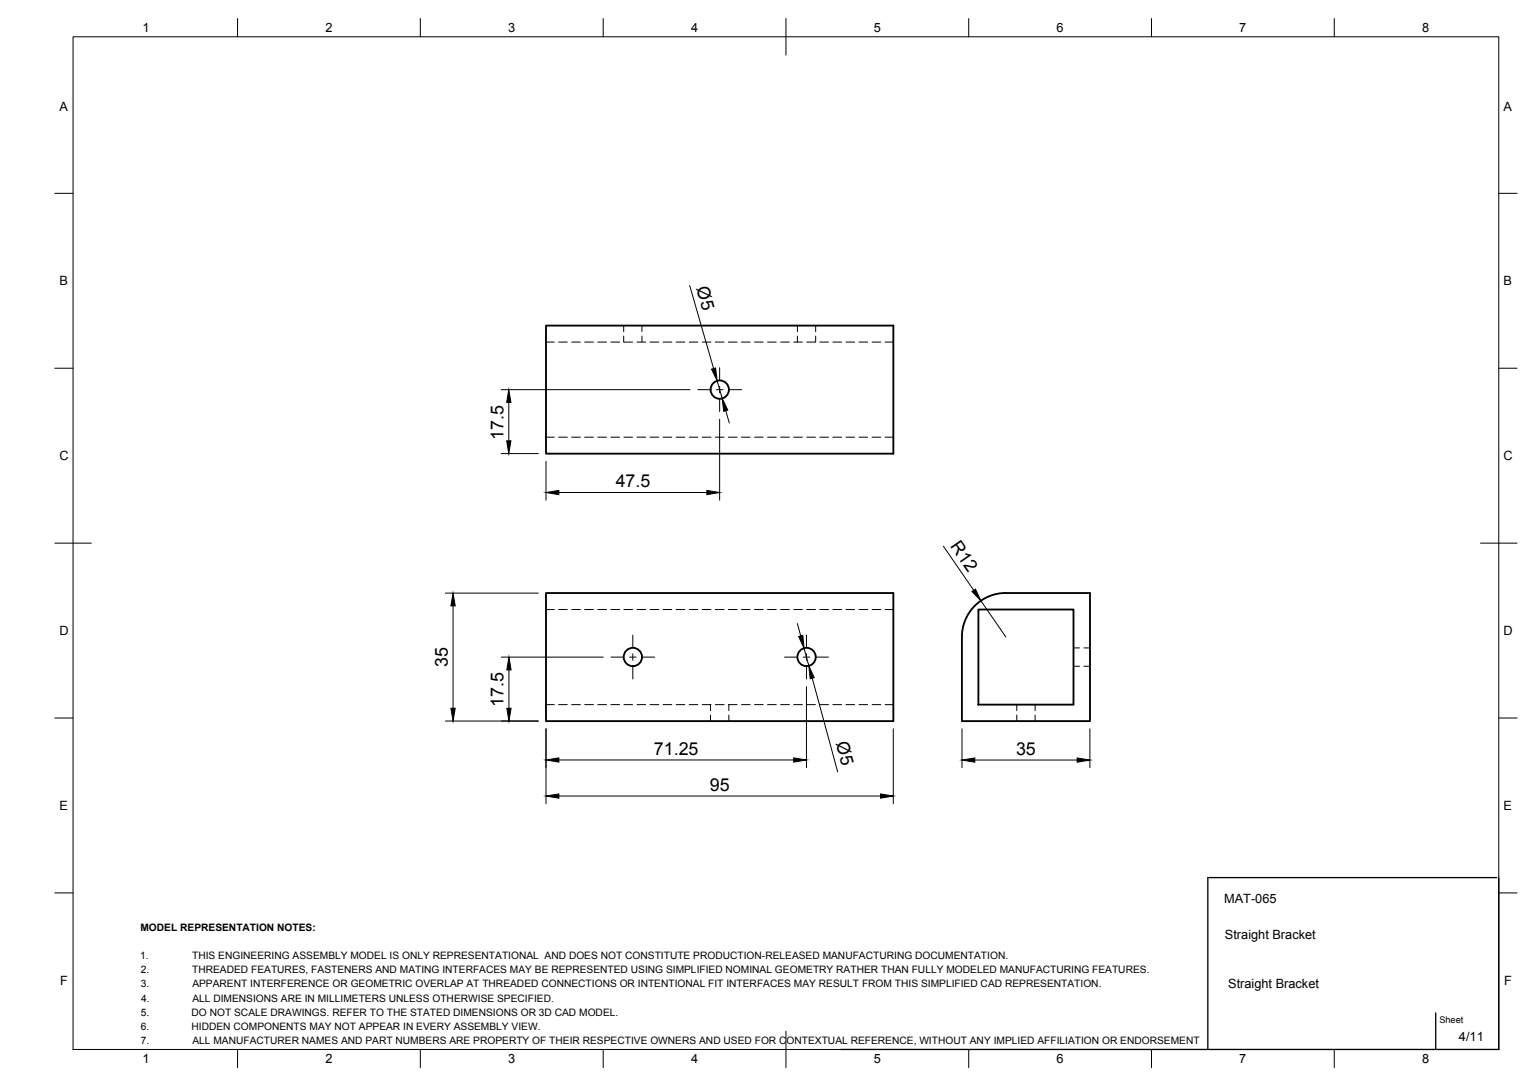
ISO-10303-21;
HEADER;
/* Generated by software containing ST-Developer
 * from STEP Tools, Inc. (www.steptools.com) 
 */

FILE_DESCRIPTION(
/* description */ (
'CAx-IF Rec.Pracs.---Representation and Presentation of Product Manufa
cturing Information (PMI)---4.0---2014-10-13'),
/* implementation_level */ '2;1');

FILE_NAME(
/* name */ 'Straight Bracket.step',
/* time_stamp */ '2026-11-15T23:28:27-08:00',
/* author */ (''),
/* organization */ (''),
/* preprocessor_version */ 'ST-DEVELOPER v20.2',
/* originating_system */ 'Autodesk Translation Framework v15.17.0.0',
/* authorisation */ '');

FILE_SCHEMA (('AUTOMOTIVE_DESIGN { 1 0 10303 214 3 1 1 }'));
ENDSEC;

DATA;
#10=MECHANICAL_DESIGN_GEOMETRIC_PRESENTATION_REPRESENTATION('',(#192),#7756);
#174=SHAPE_REPRESENTATION_RELATIONSHIP('SRR','None',#7822,#183);
#183=ADVANCED_BREP_SHAPE_REPRESENTATION('',(#201),#7750);
#192=STYLED_ITEM('',(#7876),#201);
#201=MANIFOLD_SOLID_BREP('Body1',#4629);
#216=CYLINDRICAL_SURFACE('',#4809,0.012);
#217=CYLINDRICAL_SURFACE('',#4817,0.0025);
#218=CYLINDRICAL_SURFACE('',#4818,0.0025);
#219=CYLINDRICAL_SURFACE('',#4819,0.0025);
#282=CIRCLE('',#4799,0.012);
#283=CIRCLE('',#4801,0.012);
#284=CIRCLE('',#4803,0.0025);
#285=CIRCLE('',#4806,0.0025);
#286=CIRCLE('',#4807,0.0025);
#287=CIRCLE('',#4811,0.0025);
#288=CIRCLE('',#4812,0.0025);
#289=CIRCLE('',#4814,0.0025);
#397=FACE_BOUND('',#745,.T.);
#398=FACE_BOUND('',#747,.T.);
#399=FACE_BOUND('',#749,.T.);
#400=FACE_BOUND('',#752,.T.);
#401=FACE_BOUND('',#753,.T.);
#402=FACE_BOUND('',#757,.T.);
#403=FACE_BOUND('',#758,.T.);
#404=FACE_BOUND('',#760,.T.);
#492=FACE_OUTER_BOUND('',#744,.T.);
#493=FACE_OUTER_BOUND('',#746,.T.);
#494=FACE_OUTER_BOUND('',#748,.T.);
#495=FACE_OUTER_BOUND('',#750,.T.);
#496=FACE_OUTER_BOUND('',#751,.T.);
#497=FACE_OUTER_BOUND('',#754,.T.);
#498=FACE_OUTER_BOUND('',#755,.T.);
#499=FACE_OUTER_BOUND('',#756,.T.);
#500=FACE_OUTER_BOUND('',#759,.T.);
#501=FACE_OUTER_BOUND('',#761,.T.);
#502=FACE_OUTER_BOUND('',#762,.T.);
#503=FACE_OUTER_BOUND('',#763,.T.);
#504=FACE_OUTER_BOUND('',#764,.T.);
#505=FACE_OUTER_BOUND('',#765,.T.);
#744=EDGE_LOOP('',(#3191,#3192,#3193,#3194,#3195));
#745=EDGE_LOOP('',(#3196,#3197,#3198,#3199));
#746=EDGE_LOOP('',(#3200,#3201,#3202,#3203,#3204));
#747=EDGE_LOOP('',(#3205,#3206,#3207,#3208));
#748=EDGE_LOOP('',(#3209,#3210,#3211,#3212));
#749=EDGE_LOOP('',(#3213));
#750=EDGE_LOOP('',(#3214,#3215,#3216,#3217));
#751=EDGE_LOOP('',(#3218,#3219,#3220,#3221));
#752=EDGE_LOOP('',(#3222));
#753=EDGE_LOOP('',(#3223));
#754=EDGE_LOOP('',(#3224,#3225,#3226,#3227));
#755=EDGE_LOOP('',(#3228,#3229,#3230,#3231));
#756=EDGE_LOOP('',(#3232,#3233,#3234,#3235));
#757=EDGE_LOOP('',(#3236));
#758=EDGE_LOOP('',(#3237));
#759=EDGE_LOOP('',(#3238,#3239,#3240,#3241));
#760=EDGE_LOOP('',(#3242));
#761=EDGE_LOOP('',(#3243,#3244,#3245,#3246));
#762=EDGE_LOOP('',(#3247,#3248,#3249,#3250));
#763=EDGE_LOOP('',(#3251,#3252,#3253,#3254));
#764=EDGE_LOOP('',(#3255,#3256,#3257,#3258));
#765=EDGE_LOOP('',(#3259,#3260,#3261,#3262));
#1073=LINE('',#6632,#1566);
#1074=LINE('',#6636,#1567);
#1075=LINE('',#6638,#1568);
#1076=LINE('',#6639,#1569);
#1077=LINE('',#6642,#1570);
#1078=LINE('',#6644,#1571);
#1079=LINE('',#6646,#1572);
#1080=LINE('',#6647,#1573);
#1081=LINE('',#6651,#1574);
#1082=LINE('',#6655,#1575);
#1083=LINE('',#6657,#1576);
#1084=LINE('',#6658,#1577);
#1085=LINE('',#6661,#1578);
#1086=LINE('',#6663,#1579);
#1087=LINE('',#6665,#1580);
#1088=LINE('',#6666,#1581);
#1089=LINE('',#6668,#1582);
#1090=LINE('',#6669,#1583);
#1091=LINE('',#6673,#1584);
#1092=LINE('',#6674,#1585);
#1093=LINE('',#6681,#1586);
#1094=LINE('',#6684,#1587);
#1095=LINE('',#6685,#1588);
#1096=LINE('',#6691,#1589);
#1097=LINE('',#6695,#1590);
#1098=LINE('',#6698,#1591);
#1099=LINE('',#6700,#1592);
#1100=LINE('',#6702,#1593);
#1566=VECTOR('',#5341,1.);
#1567=VECTOR('',#5344,1.);
#1568=VECTOR('',#5345,1.);
#1569=VECTOR('',#5346,1.);
#1570=VECTOR('',#5347,1.);
#1571=VECTOR('',#5348,1.);
#1572=VECTOR('',#5349,1.);
#1573=VECTOR('',#5350,1.);
#1574=VECTOR('',#5353,1.);
#1575=VECTOR('',#5356,1.);
#1576=VECTOR('',#5357,1.);
#1577=VECTOR('',#5358,1.);
#1578=VECTOR('',#5359,1.);
#1579=VECTOR('',#5360,1.);
#1580=VECTOR('',#5361,1.);
#1581=VECTOR('',#5362,1.);
#1582=VECTOR('',#5365,1.);
#1583=VECTOR('',#5366,1.);
#1584=VECTOR('',#5371,1.);
#1585=VECTOR('',#5372,1.);
#1586=VECTOR('',#5381,1.);
#1587=VECTOR('',#5386,1.);
#1588=VECTOR('',#5387,1.);
#1589=VECTOR('',#5394,1.);
#1590=VECTOR('',#5399,1.);
#1591=VECTOR('',#5404,0.0025);
#1592=VECTOR('',#5407,0.0025);
#1593=VECTOR('',#5410,0.0025);
#2044=VERTEX_POINT('',#6630);
#2045=VERTEX_POINT('',#6631);
#2046=VERTEX_POINT('',#6633);
#2047=VERTEX_POINT('',#6635);
#2048=VERTEX_POINT('',#6637);
#2049=VERTEX_POINT('',#6640);
#2050=VERTEX_POINT('',#6641);
#2051=VERTEX_POINT('',#6643);
#2052=VERTEX_POINT('',#6645);
#2053=VERTEX_POINT('',#6649);
#2054=VERTEX_POINT('',#6650);
#2055=VERTEX_POINT('',#6652);
#2056=VERTEX_POINT('',#6654);
#2057=VERTEX_POINT('',#6656);
#2058=VERTEX_POINT('',#6659);
#2059=VERTEX_POINT('',#6660);
#2060=VERTEX_POINT('',#6662);
#2061=VERTEX_POINT('',#6664);
#2062=VERTEX_POINT('',#6670);
#2063=VERTEX_POINT('',#6676);
#2064=VERTEX_POINT('',#6678);
#2065=VERTEX_POINT('',#6686);
#2066=VERTEX_POINT('',#6688);
#2067=VERTEX_POINT('',#6692);
#2479=EDGE_CURVE('',#2044,#2045,#1073,.T.);
#2480=EDGE_CURVE('',#2045,#2046,#282,.F.);
#2481=EDGE_CURVE('',#2047,#2046,#1074,.T.);
#2482=EDGE_CURVE('',#2048,#2047,#1075,.T.);
#2483=EDGE_CURVE('',#2048,#2044,#1076,.T.);
#2484=EDGE_CURVE('',#2049,#2050,#1077,.T.);
#2485=EDGE_CURVE('',#2050,#2051,#1078,.T.);
#2486=EDGE_CURVE('',#2052,#2051,#1079,.T.);
#2487=EDGE_CURVE('',#2049,#2052,#1080,.T.);
#2488=EDGE_CURVE('',#2053,#2054,#1081,.T.);
#2489=EDGE_CURVE('',#2054,#2055,#283,.T.);
#2490=EDGE_CURVE('',#2056,#2055,#1082,.T.);
#2491=EDGE_CURVE('',#2057,#2056,#1083,.T.);
#2492=EDGE_CURVE('',#2057,#2053,#1084,.T.);
#2493=EDGE_CURVE('',#2058,#2059,#1085,.T.);
#2494=EDGE_CURVE('',#2059,#2060,#1086,.T.);
#2495=EDGE_CURVE('',#2061,#2060,#1087,.T.);
#2496=EDGE_CURVE('',#2058,#2061,#1088,.T.);
#2497=EDGE_CURVE('',#2044,#2056,#1089,.T.);
#2498=EDGE_CURVE('',#2048,#2057,#1090,.T.);
#2499=EDGE_CURVE('',#2062,#2062,#284,.T.);
#2500=EDGE_CURVE('',#2046,#2054,#1091,.T.);
#2501=EDGE_CURVE('',#2047,#2053,#1092,.T.);
#2502=EDGE_CURVE('',#2063,#2063,#285,.T.);
#2503=EDGE_CURVE('',#2064,#2064,#286,.T.);
#2504=EDGE_CURVE('',#2055,#2045,#1093,.F.);
#2505=EDGE_CURVE('',#2059,#2050,#1094,.T.);
#2506=EDGE_CURVE('',#2060,#2049,#1095,.T.);
#2507=EDGE_CURVE('',#2065,#2065,#287,.T.);
#2508=EDGE_CURVE('',#2066,#2066,#288,.T.);
#2509=EDGE_CURVE('',#2061,#2052,#1096,.T.);
#2510=EDGE_CURVE('',#2067,#2067,#289,.T.);
#2511=EDGE_CURVE('',#2058,#2051,#1097,.T.);
#2512=EDGE_CURVE('',#2067,#2062,#1098,.T.);
#2513=EDGE_CURVE('',#2066,#2064,#1099,.T.);
#2514=EDGE_CURVE('',#2065,#2063,#1100,.T.);
#3191=ORIENTED_EDGE('',*,*,#2479,.T.);
#3192=ORIENTED_EDGE('',*,*,#2480,.T.);
#3193=ORIENTED_EDGE('',*,*,#2481,.F.);
#3194=ORIENTED_EDGE('',*,*,#2482,.F.);
#3195=ORIENTED_EDGE('',*,*,#2483,.T.);
#3196=ORIENTED_EDGE('',*,*,#2484,.T.);
#3197=ORIENTED_EDGE('',*,*,#2485,.T.);
#3198=ORIENTED_EDGE('',*,*,#2486,.F.);
#3199=ORIENTED_EDGE('',*,*,#2487,.F.);
#3200=ORIENTED_EDGE('',*,*,#2488,.T.);
#3201=ORIENTED_EDGE('',*,*,#2489,.T.);
#3202=ORIENTED_EDGE('',*,*,#2490,.F.);
#3203=ORIENTED_EDGE('',*,*,#2491,.F.);
#3204=ORIENTED_EDGE('',*,*,#2492,.T.);
#3205=ORIENTED_EDGE('',*,*,#2493,.T.);
#3206=ORIENTED_EDGE('',*,*,#2494,.T.);
#3207=ORIENTED_EDGE('',*,*,#2495,.F.);
#3208=ORIENTED_EDGE('',*,*,#2496,.F.);
#3209=ORIENTED_EDGE('',*,*,#2497,.F.);
#3210=ORIENTED_EDGE('',*,*,#2483,.F.);
#3211=ORIENTED_EDGE('',*,*,#2498,.T.);
#3212=ORIENTED_EDGE('',*,*,#2491,.T.);
#3213=ORIENTED_EDGE('',*,*,#2499,.F.);
#3214=ORIENTED_EDGE('',*,*,#2481,.T.);
#3215=ORIENTED_EDGE('',*,*,#2500,.T.);
#3216=ORIENTED_EDGE('',*,*,#2488,.F.);
#3217=ORIENTED_EDGE('',*,*,#2501,.F.);
#3218=ORIENTED_EDGE('',*,*,#2498,.F.);
#3219=ORIENTED_EDGE('',*,*,#2482,.T.);
#3220=ORIENTED_EDGE('',*,*,#2501,.T.);
#3221=ORIENTED_EDGE('',*,*,#2492,.F.);
#3222=ORIENTED_EDGE('',*,*,#2502,.F.);
#3223=ORIENTED_EDGE('',*,*,#2503,.F.);
#3224=ORIENTED_EDGE('',*,*,#2490,.T.);
#3225=ORIENTED_EDGE('',*,*,#2504,.T.);
#3226=ORIENTED_EDGE('',*,*,#2479,.F.);
#3227=ORIENTED_EDGE('',*,*,#2497,.T.);
#3228=ORIENTED_EDGE('',*,*,#2480,.F.);
#3229=ORIENTED_EDGE('',*,*,#2504,.F.);
#3230=ORIENTED_EDGE('',*,*,#2489,.F.);
#3231=ORIENTED_EDGE('',*,*,#2500,.F.);
#3232=ORIENTED_EDGE('',*,*,#2505,.T.);
#3233=ORIENTED_EDGE('',*,*,#2484,.F.);
#3234=ORIENTED_EDGE('',*,*,#2506,.F.);
#3235=ORIENTED_EDGE('',*,*,#2494,.F.);
#3236=ORIENTED_EDGE('',*,*,#2507,.F.);
#3237=ORIENTED_EDGE('',*,*,#2508,.F.);
#3238=ORIENTED_EDGE('',*,*,#2495,.T.);
#3239=ORIENTED_EDGE('',*,*,#2506,.T.);
#3240=ORIENTED_EDGE('',*,*,#2487,.T.);
#3241=ORIENTED_EDGE('',*,*,#2509,.F.);
#3242=ORIENTED_EDGE('',*,*,#2510,.T.);
#3243=ORIENTED_EDGE('',*,*,#2496,.T.);
#3244=ORIENTED_EDGE('',*,*,#2509,.T.);
#3245=ORIENTED_EDGE('',*,*,#2486,.T.);
#3246=ORIENTED_EDGE('',*,*,#2511,.F.);
#3247=ORIENTED_EDGE('',*,*,#2511,.T.);
#3248=ORIENTED_EDGE('',*,*,#2485,.F.);
#3249=ORIENTED_EDGE('',*,*,#2505,.F.);
#3250=ORIENTED_EDGE('',*,*,#2493,.F.);
#3251=ORIENTED_EDGE('',*,*,#2510,.F.);
#3252=ORIENTED_EDGE('',*,*,#2512,.T.);
#3253=ORIENTED_EDGE('',*,*,#2499,.T.);
#3254=ORIENTED_EDGE('',*,*,#2512,.F.);
#3255=ORIENTED_EDGE('',*,*,#2508,.T.);
#3256=ORIENTED_EDGE('',*,*,#2513,.T.);
#3257=ORIENTED_EDGE('',*,*,#2503,.T.);
#3258=ORIENTED_EDGE('',*,*,#2513,.F.);
#3259=ORIENTED_EDGE('',*,*,#2507,.T.);
#3260=ORIENTED_EDGE('',*,*,#2514,.T.);
#3261=ORIENTED_EDGE('',*,*,#2502,.T.);
#3262=ORIENTED_EDGE('',*,*,#2514,.F.);
#4250=PLANE('',#4798);
#4251=PLANE('',#4800);
#4252=PLANE('',#4802);
#4253=PLANE('',#4804);
#4254=PLANE('',#4805);
#4255=PLANE('',#4808);
#4256=PLANE('',#4810);
#4257=PLANE('',#4813);
#4258=PLANE('',#4815);
#4259=PLANE('',#4816);
#4433=ADVANCED_FACE('',(#492,#397),#4250,.F.);
#4434=ADVANCED_FACE('',(#493,#398),#4251,.T.);
#4435=ADVANCED_FACE('',(#494,#399),#4252,.T.);
#4436=ADVANCED_FACE('',(#495),#4253,.F.);
#4437=ADVANCED_FACE('',(#496,#400,#401),#4254,.T.);
#4438=ADVANCED_FACE('',(#497),#4255,.F.);
#4439=ADVANCED_FACE('',(#498),#216,.T.);
#4440=ADVANCED_FACE('',(#499,#402,#403),#4256,.T.);
#4441=ADVANCED_FACE('',(#500,#404),#4257,.F.);
#4442=ADVANCED_FACE('',(#501),#4258,.F.);
#4443=ADVANCED_FACE('',(#502),#4259,.T.);
#4444=ADVANCED_FACE('',(#503),#217,.F.);
#4445=ADVANCED_FACE('',(#504),#218,.F.);
#4446=ADVANCED_FACE('',(#505),#219,.F.);
#4629=CLOSED_SHELL('',(#4433,#4434,#4435,#4436,#4437,#4438,#4439,#4440,
#4441,#4442,#4443,#4444,#4445,#4446));
#4797=AXIS2_PLACEMENT_3D('',#6628,#5337,#5338);
#4798=AXIS2_PLACEMENT_3D('',#6629,#5339,#5340);
#4799=AXIS2_PLACEMENT_3D('',#6634,#5342,#5343);
#4800=AXIS2_PLACEMENT_3D('',#6648,#5351,#5352);
#4801=AXIS2_PLACEMENT_3D('',#6653,#5354,#5355);
#4802=AXIS2_PLACEMENT_3D('',#6667,#5363,#5364);
#4803=AXIS2_PLACEMENT_3D('',#6671,#5367,#5368);
#4804=AXIS2_PLACEMENT_3D('',#6672,#5369,#5370);
#4805=AXIS2_PLACEMENT_3D('',#6675,#5373,#5374);
#4806=AXIS2_PLACEMENT_3D('',#6677,#5375,#5376);
#4807=AXIS2_PLACEMENT_3D('',#6679,#5377,#5378);
#4808=AXIS2_PLACEMENT_3D('',#6680,#5379,#5380);
#4809=AXIS2_PLACEMENT_3D('',#6682,#5382,#5383);
#4810=AXIS2_PLACEMENT_3D('',#6683,#5384,#5385);
#4811=AXIS2_PLACEMENT_3D('',#6687,#5388,#5389);
#4812=AXIS2_PLACEMENT_3D('',#6689,#5390,#5391);
#4813=AXIS2_PLACEMENT_3D('',#6690,#5392,#5393);
#4814=AXIS2_PLACEMENT_3D('',#6693,#5395,#5396);
#4815=AXIS2_PLACEMENT_3D('',#6694,#5397,#5398);
#4816=AXIS2_PLACEMENT_3D('',#6696,#5400,#5401);
#4817=AXIS2_PLACEMENT_3D('',#6697,#5402,#5403);
#4818=AXIS2_PLACEMENT_3D('',#6699,#5405,#5406);
#4819=AXIS2_PLACEMENT_3D('',#6701,#5408,#5409);
#5337=DIRECTION('axis',(0.,0.,1.));
#5338=DIRECTION('refdir',(1.,0.,0.));
#5339=DIRECTION('center_axis',(1.,0.,0.));
#5340=DIRECTION('ref_axis',(0.,0.,-1.));
#5341=DIRECTION('',(0.,-1.,0.));
#5342=DIRECTION('center_axis',(1.,0.,0.));
#5343=DIRECTION('ref_axis',(0.,0.,-1.));
#5344=DIRECTION('',(0.,0.,-1.));
#5345=DIRECTION('',(0.,-1.,0.));
#5346=DIRECTION('',(0.,0.,-1.));
#5347=DIRECTION('',(0.,-1.,0.));
#5348=DIRECTION('',(0.,0.,-1.));
#5349=DIRECTION('',(0.,-1.,0.));
#5350=DIRECTION('',(0.,-6.67201336914157E-17,-1.));
#5351=DIRECTION('center_axis',(1.,0.,0.));
#5352=DIRECTION('ref_axis',(0.,0.,-1.));
#5353=DIRECTION('',(0.,0.,-1.));
#5354=DIRECTION('center_axis',(1.,0.,0.));
#5355=DIRECTION('ref_axis',(0.,0.,-1.));
#5356=DIRECTION('',(0.,-1.,0.));
#5357=DIRECTION('',(0.,0.,-1.));
#5358=DIRECTION('',(0.,-1.,0.));
#5359=DIRECTION('',(0.,0.,1.));
#5360=DIRECTION('',(0.,1.,0.));
#5361=DIRECTION('',(0.,6.67201336914157E-17,1.));
#5362=DIRECTION('',(0.,1.,0.));
#5363=DIRECTION('center_axis',(-1.82602471155453E-16,1.,0.));
#5364=DIRECTION('ref_axis',(-1.,-1.82602471155453E-16,0.));
#5365=DIRECTION('',(1.,1.82602471155453E-16,0.));
#5366=DIRECTION('',(1.,1.82602471155453E-16,0.));
#5367=DIRECTION('center_axis',(-1.82602471155453E-16,1.,0.));
#5368=DIRECTION('ref_axis',(-1.,-1.82602471155453E-16,0.));
#5369=DIRECTION('center_axis',(-2.19122965386544E-16,1.,0.));
#5370=DIRECTION('ref_axis',(-1.,-2.19122965386544E-16,0.));
#5371=DIRECTION('',(1.,2.19122965386544E-16,0.));
#5372=DIRECTION('',(1.,2.19122965386544E-16,0.));
#5373=DIRECTION('center_axis',(0.,0.,1.));
#5374=DIRECTION('ref_axis',(1.,0.,0.));
#5375=DIRECTION('center_axis',(0.,0.,1.));
#5376=DIRECTION('ref_axis',(1.,0.,0.));
#5377=DIRECTION('center_axis',(0.,0.,1.));
#5378=DIRECTION('ref_axis',(1.,0.,0.));
#5379=DIRECTION('center_axis',(0.,0.,1.));
#5380=DIRECTION('ref_axis',(1.,0.,0.));
#5381=DIRECTION('',(1.,2.19122965386544E-16,0.));
#5382=DIRECTION('center_axis',(1.,2.19122965386544E-16,0.));
#5383=DIRECTION('ref_axis',(-2.19122965386544E-16,1.,0.));
#5384=DIRECTION('center_axis',(0.,0.,-1.));
#5385=DIRECTION('ref_axis',(-1.,0.,0.));
#5386=DIRECTION('',(-1.,0.,0.));
#5387=DIRECTION('',(-1.,0.,0.));
#5388=DIRECTION('center_axis',(0.,0.,-1.));
#5389=DIRECTION('ref_axis',(-1.,0.,0.));
#5390=DIRECTION('center_axis',(0.,0.,-1.));
#5391=DIRECTION('ref_axis',(-1.,0.,0.));
#5392=DIRECTION('center_axis',(0.,1.,-6.67201336914157E-17));
#5393=DIRECTION('ref_axis',(0.,6.67201336914157E-17,1.));
#5394=DIRECTION('',(-1.,0.,0.));
#5395=DIRECTION('center_axis',(0.,1.,-6.67201336914157E-17));
#5396=DIRECTION('ref_axis',(0.,6.67201336914157E-17,1.));
#5397=DIRECTION('center_axis',(0.,0.,-1.));
#5398=DIRECTION('ref_axis',(-1.,0.,0.));
#5399=DIRECTION('',(-1.,0.,0.));
#5400=DIRECTION('center_axis',(0.,1.,0.));
#5401=DIRECTION('ref_axis',(0.,0.,1.));
#5402=DIRECTION('center_axis',(-1.82602471155453E-16,1.,0.));
#5403=DIRECTION('ref_axis',(-1.,-1.82602471155453E-16,0.));
#5404=DIRECTION('',(-1.82602471155453E-16,1.,0.));
#5405=DIRECTION('center_axis',(0.,0.,1.));
#5406=DIRECTION('ref_axis',(1.,0.,0.));
#5407=DIRECTION('',(0.,0.,1.));
#5408=DIRECTION('center_axis',(0.,0.,1.));
#5409=DIRECTION('ref_axis',(1.,0.,0.));
#5410=DIRECTION('',(0.,0.,1.));
#6628=CARTESIAN_POINT('',(0.,0.,0.));
#6629=CARTESIAN_POINT('Origin',(-0.0475,-1.04083408558608E-17,0.035));
#6630=CARTESIAN_POINT('',(-0.0475,0.0175,0.));
#6631=CARTESIAN_POINT('',(-0.0475,-0.0055,0.));
#6632=CARTESIAN_POINT('',(-0.0475,-1.04083408558608E-17,0.));
#6633=CARTESIAN_POINT('',(-0.0475,-0.0175,0.012));
#6634=CARTESIAN_POINT('Origin',(-0.0475,-0.0055,0.012));
#6635=CARTESIAN_POINT('',(-0.0475,-0.0175,0.035));
#6636=CARTESIAN_POINT('',(-0.0475,-0.0175,0.035));
#6637=CARTESIAN_POINT('',(-0.0475,0.0175,0.035));
#6638=CARTESIAN_POINT('',(-0.0475,-1.04083408558608E-17,0.035));
#6639=CARTESIAN_POINT('',(-0.0475,0.0175,0.035));
#6640=CARTESIAN_POINT('',(-0.0475,0.013,0.0305));
#6641=CARTESIAN_POINT('',(-0.0475,-0.013,0.0305));
#6642=CARTESIAN_POINT('',(-0.0475,-1.04083408558608E-17,0.0305));
#6643=CARTESIAN_POINT('',(-0.0475,-0.013,0.0045));
#6644=CARTESIAN_POINT('',(-0.0475,-0.013,0.0175));
#6645=CARTESIAN_POINT('',(-0.0475,0.013,0.0045));
#6646=CARTESIAN_POINT('',(-0.0475,-1.21430643318376E-17,0.0045));
#6647=CARTESIAN_POINT('',(-0.0475,0.013,0.0175));
#6648=CARTESIAN_POINT('Origin',(0.0475,6.93889390390723E-18,0.035));
#6649=CARTESIAN_POINT('',(0.0475,-0.0175,0.035));
#6650=CARTESIAN_POINT('',(0.0475,-0.0175,0.012));
#6651=CARTESIAN_POINT('',(0.0475,-0.0175,0.035));
#6652=CARTESIAN_POINT('',(0.0475,-0.0055,0.));
#6653=CARTESIAN_POINT('Origin',(0.0475,-0.0055,0.012));
#6654=CARTESIAN_POINT('',(0.0475,0.0175,0.));
#6655=CARTESIAN_POINT('',(0.0475,6.93889390390723E-18,0.));
#6656=CARTESIAN_POINT('',(0.0475,0.0175,0.035));
#6657=CARTESIAN_POINT('',(0.0475,0.0175,0.035));
#6658=CARTESIAN_POINT('',(0.0475,6.93889390390723E-18,0.035));
#6659=CARTESIAN_POINT('',(0.0475,-0.013,0.0045));
#6660=CARTESIAN_POINT('',(0.0475,-0.013,0.0305));
#6661=CARTESIAN_POINT('',(0.0475,-0.013,0.035));
#6662=CARTESIAN_POINT('',(0.0475,0.013,0.0305));
#6663=CARTESIAN_POINT('',(0.0475,6.93889390390723E-18,0.0305));
#6664=CARTESIAN_POINT('',(0.0475,0.013,0.0045));
#6665=CARTESIAN_POINT('',(0.0475,0.013,0.035));
#6666=CARTESIAN_POINT('',(0.0475,6.93889390390723E-18,0.0045));
#6667=CARTESIAN_POINT('Origin',(6.93889390390723E-18,0.0175,0.035));
#6668=CARTESIAN_POINT('',(6.93889390390723E-18,0.0175,0.));
#6669=CARTESIAN_POINT('',(6.93889390390723E-18,0.0175,0.035));
#6670=CARTESIAN_POINT('',(0.0025,0.0175,0.0175));
#6671=CARTESIAN_POINT('Origin',(-3.46944695195361E-18,0.0175,0.0175));
#6672=CARTESIAN_POINT('Origin',(6.93889390390723E-18,-0.0175,0.035));
#6673=CARTESIAN_POINT('',(6.93889390390723E-18,-0.0175,0.012));
#6674=CARTESIAN_POINT('',(6.93889390390723E-18,-0.0175,0.035));
#6675=CARTESIAN_POINT('Origin',(6.93889390390723E-18,0.,0.035));
#6676=CARTESIAN_POINT('',(-0.02625,-1.53080849893419E-19,0.035));
#6677=CARTESIAN_POINT('Origin',(-0.02375,1.53080849893419E-19,0.035));
#6678=CARTESIAN_POINT('',(0.02125,-3.06161699786838E-19,0.035));
#6679=CARTESIAN_POINT('Origin',(0.02375,-4.81482486096809E-35,0.035));
#6680=CARTESIAN_POINT('Origin',(6.93889390390723E-18,0.,0.));
#6681=CARTESIAN_POINT('',(8.14407021353322E-18,-0.0055,0.));
#6682=CARTESIAN_POINT('Origin',(4.3094183192687E-18,-0.0055,0.012));
#6683=CARTESIAN_POINT('Origin',(0.0525,-1.04083408558608E-17,0.0305));
#6684=CARTESIAN_POINT('',(0.0525,-0.013,0.0305));
#6685=CARTESIAN_POINT('',(0.0525,0.013,0.0305));
#6686=CARTESIAN_POINT('',(-0.02625,1.53080849893419E-19,0.0305));
#6687=CARTESIAN_POINT('Origin',(-0.02375,1.53080849893419E-19,0.0305));
#6688=CARTESIAN_POINT('',(0.02125,-4.81482486096809E-35,0.0305));
#6689=CARTESIAN_POINT('Origin',(0.02375,-4.81482486096809E-35,0.0305));
#6690=CARTESIAN_POINT('Origin',(0.0525,0.013,0.0175));
#6691=CARTESIAN_POINT('',(0.0525,0.013,0.0045));
#6692=CARTESIAN_POINT('',(0.0025,0.013,0.0175));
#6693=CARTESIAN_POINT('Origin',(-2.64773583175407E-18,0.013,0.0175));
#6694=CARTESIAN_POINT('Origin',(0.0525,-1.21430643318376E-17,0.0045));
#6695=CARTESIAN_POINT('',(0.0525,-0.013,0.0045));
#6696=CARTESIAN_POINT('Origin',(0.0525,-0.013,0.0175));
#6697=CARTESIAN_POINT('Origin',(-1.64342224039908E-18,0.0075,0.0175));
#6698=CARTESIAN_POINT('',(0.0025,0.0075,0.0175));
#6699=CARTESIAN_POINT('Origin',(0.02375,-4.81482486096809E-35,0.025));
#6700=CARTESIAN_POINT('',(0.02125,-3.06161699786838E-19,0.025));
#6701=CARTESIAN_POINT('Origin',(-0.02375,1.53080849893419E-19,0.025));
#6702=CARTESIAN_POINT('',(-0.02625,-1.53080849893419E-19,0.025));
#7739=UNCERTAINTY_MEASURE_WITH_UNIT(LENGTH_MEASURE(1.E-5),#7757,
'DISTANCE_ACCURACY_VALUE',
'Maximum model space distance between geometric entities at asserted c
onnectivities');
#7745=UNCERTAINTY_MEASURE_WITH_UNIT(LENGTH_MEASURE(1.E-5),#7757,
'DISTANCE_ACCURACY_VALUE',
'Maximum model space distance between geometric entities at asserted c
onnectivities');
#7750=(
GEOMETRIC_REPRESENTATION_CONTEXT(3)
GLOBAL_UNCERTAINTY_ASSIGNED_CONTEXT((#7739))
GLOBAL_UNIT_ASSIGNED_CONTEXT((#7757,#7758,#7759))
REPRESENTATION_CONTEXT('','3D')
);
#7756=(
GEOMETRIC_REPRESENTATION_CONTEXT(3)
GLOBAL_UNCERTAINTY_ASSIGNED_CONTEXT((#7745))
GLOBAL_UNIT_ASSIGNED_CONTEXT((#7757,#7758,#7759))
REPRESENTATION_CONTEXT('','3D')
);
#7757=(
LENGTH_UNIT()
NAMED_UNIT(*)
SI_UNIT($,.METRE.)
);
#7758=(
NAMED_UNIT(*)
PLANE_ANGLE_UNIT()
SI_UNIT($,.RADIAN.)
);
#7759=(
NAMED_UNIT(*)
SI_UNIT($,.STERADIAN.)
SOLID_ANGLE_UNIT()
);
#7764=SHAPE_DEFINITION_REPRESENTATION(#7774,#7822);
#7774=PRODUCT_DEFINITION_SHAPE('',$,#7833);
#7822=SHAPE_REPRESENTATION('',(#4797),#7750);
#7828=PRODUCT_DEFINITION_CONTEXT('part definition',#7860,'design');
#7833=PRODUCT_DEFINITION('Straight Bracket','Straight Bracket',#7843,#7828);
#7843=PRODUCT_DEFINITION_FORMATION('',$,#7866);
#7860=APPLICATION_CONTEXT(
'Core Data for Automotive Mechanical Design Process');
#7861=PRODUCT_CONTEXT('part definition',#7860,'mechanical');
#7866=PRODUCT('Straight Bracket','Straight Bracket',
'LEGAL AND USAGE DISCLAIMER: this Data/Model is provided \X2\201C\X0\A
S IS\X2\201D\X0\ for informational and representational only. It is a 
geometric approximation and is NOT engineered, certified, or guarantee
d for dimensional accuracy, exact tolerances, or production-level prec
ision. Vendor disclaims all implied warranties including fitness for a
 particular purpose. DO NOT USE FOR DIRECT PHYSICAL MANUFACTURING, AUT
OMATED PRODUCTION, OR SAFETY-CRITICAL SYSTEMS without independent engi
neering verification and resolution of any design discrepancies.',(#7861));
#7876=PRESENTATION_STYLE_ASSIGNMENT((#7883));
#7883=SURFACE_STYLE_USAGE(.BOTH.,#7890);
#7890=SURFACE_SIDE_STYLE('',(#7897));
#7897=SURFACE_STYLE_FILL_AREA(#7904);
#7904=FILL_AREA_STYLE('Opaque(137,137,137)',(#7911));
#7911=FILL_AREA_STYLE_COLOUR('Opaque(137,137,137)',#7918);
#7918=COLOUR_RGB('Opaque(137,137,137)',0.537254901960784,0.537254901960784,
0.537254901960784);
ENDSEC;
END-ISO-10303-21;
